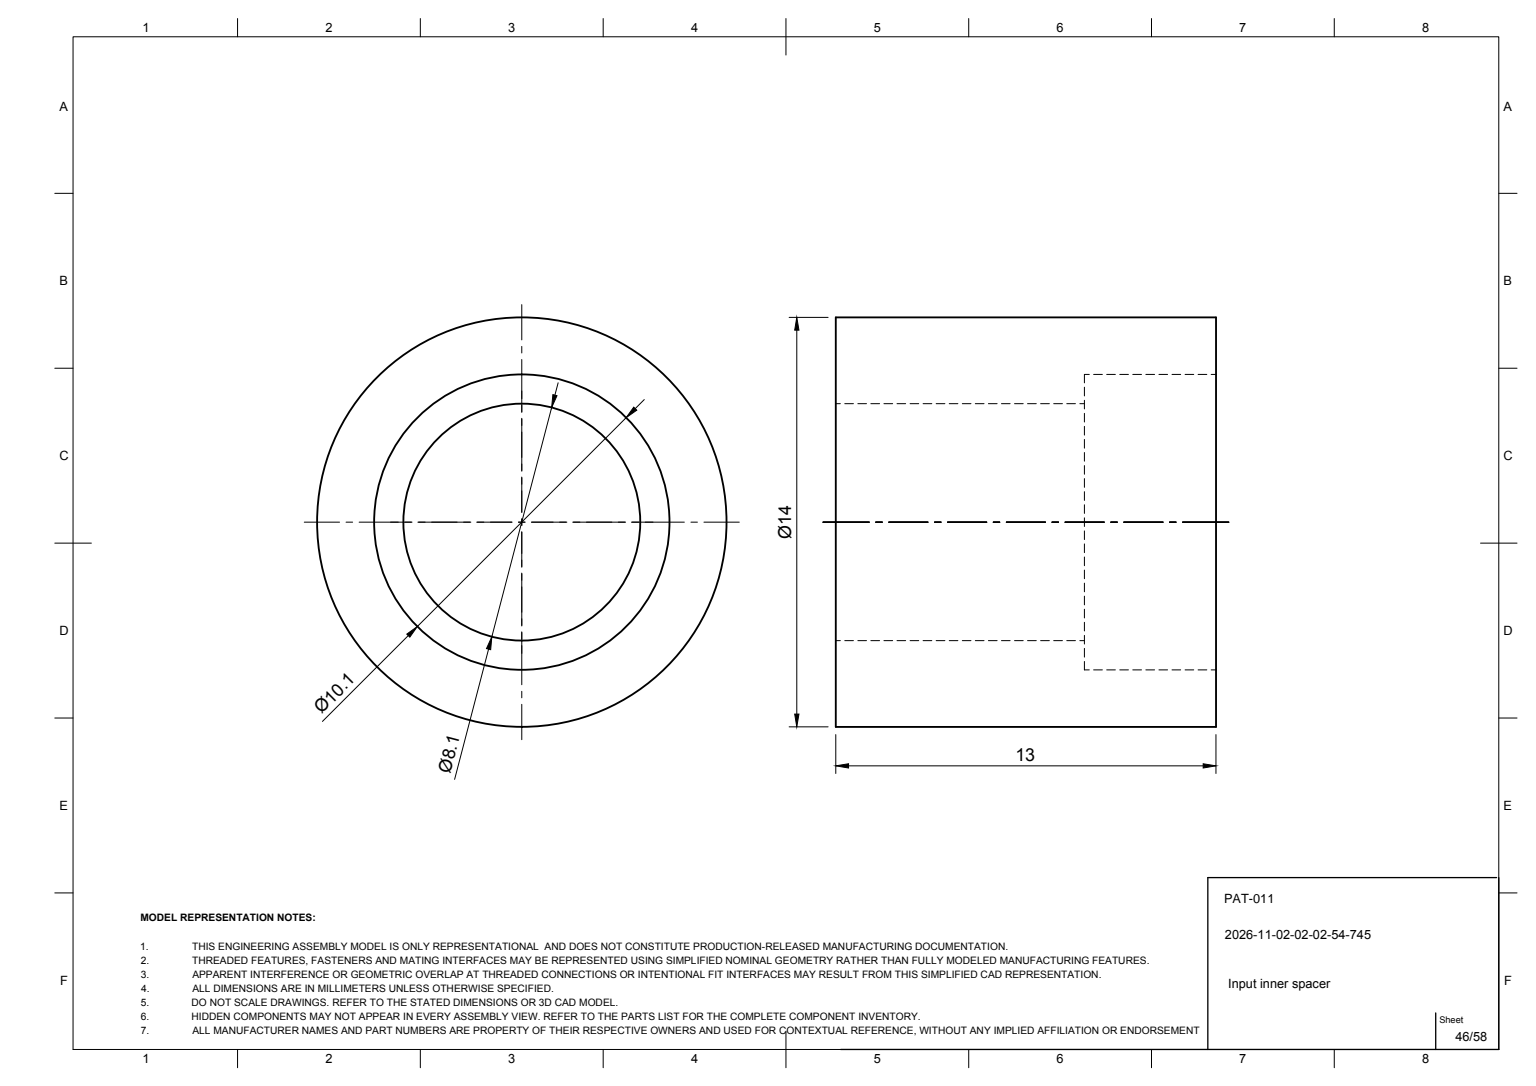
ISO-10303-21;
HEADER;
/* Generated by software containing ST-Developer
 * from STEP Tools, Inc. (www.steptools.com) 
 */

FILE_DESCRIPTION(
/* description */ ('Belt tension measurement rig'),
/* implementation_level */ '2;1');

FILE_NAME(
/* name */ 'Input inner spacer.step',
/* time_stamp */ '2026-10-28T03:24:44-07:00',
/* author */ (''),
/* organization */ (''),
/* preprocessor_version */ 'ST-DEVELOPER v20.2',
/* originating_system */ 'Autodesk Translation Framework v15.17.0.0',
/* authorisation */ '');

FILE_SCHEMA (('AUTOMOTIVE_DESIGN { 1 0 10303 214 3 1 1 }'));
ENDSEC;

DATA;
#10=MECHANICAL_DESIGN_GEOMETRIC_PRESENTATION_REPRESENTATION('',(#745),#23587);
#620=SHAPE_REPRESENTATION_RELATIONSHIP('SRR','None',#23870,#675);
#675=ADVANCED_BREP_SHAPE_REPRESENTATION('',(#813),#23568);
#745=STYLED_ITEM('',(#24225),#813);
#813=MANIFOLD_SOLID_BREP('Body1',#12252);
#988=FACE_BOUND('',#2675,.T.);
#989=FACE_BOUND('',#2679,.T.);
#990=FACE_BOUND('',#2681,.T.);
#1283=PLANE('',#13832);
#1284=PLANE('',#13839);
#1285=PLANE('',#13840);
#1810=FACE_OUTER_BOUND('',#2673,.T.);
#1811=FACE_OUTER_BOUND('',#2674,.T.);
#1812=FACE_OUTER_BOUND('',#2676,.T.);
#1813=FACE_OUTER_BOUND('',#2677,.T.);
#1814=FACE_OUTER_BOUND('',#2678,.T.);
#1815=FACE_OUTER_BOUND('',#2680,.T.);
#2673=EDGE_LOOP('',(#9950,#9951,#9952,#9953));
#2674=EDGE_LOOP('',(#9954));
#2675=EDGE_LOOP('',(#9955));
#2676=EDGE_LOOP('',(#9956,#9957,#9958,#9959));
#2677=EDGE_LOOP('',(#9960,#9961,#9962,#9963));
#2678=EDGE_LOOP('',(#9964));
#2679=EDGE_LOOP('',(#9965));
#2680=EDGE_LOOP('',(#9966));
#2681=EDGE_LOOP('',(#9967));
#3498=LINE('',#21484,#4249);
#3499=LINE('',#21491,#4250);
#3500=LINE('',#21497,#4251);
#4249=VECTOR('',#16957,0.505);
#4250=VECTOR('',#16966,0.405);
#4251=VECTOR('',#16973,0.7);
#4906=CIRCLE('',#13830,0.505);
#4907=CIRCLE('',#13831,0.505);
#4908=CIRCLE('',#13833,0.405);
#4909=CIRCLE('',#13835,0.405);
#4910=CIRCLE('',#13837,0.7);
#4911=CIRCLE('',#13838,0.7);
#5921=VERTEX_POINT('',#21481);
#5922=VERTEX_POINT('',#21483);
#5923=VERTEX_POINT('',#21487);
#5924=VERTEX_POINT('',#21490);
#5925=VERTEX_POINT('',#21494);
#5926=VERTEX_POINT('',#21496);
#7334=EDGE_CURVE('',#5921,#5921,#4906,.T.);
#7335=EDGE_CURVE('',#5921,#5922,#3498,.T.);
#7336=EDGE_CURVE('',#5922,#5922,#4907,.T.);
#7337=EDGE_CURVE('',#5923,#5923,#4908,.T.);
#7338=EDGE_CURVE('',#5923,#5924,#3499,.T.);
#7339=EDGE_CURVE('',#5924,#5924,#4909,.T.);
#7340=EDGE_CURVE('',#5925,#5925,#4910,.T.);
#7341=EDGE_CURVE('',#5925,#5926,#3500,.T.);
#7342=EDGE_CURVE('',#5926,#5926,#4911,.T.);
#9950=ORIENTED_EDGE('',*,*,#7334,.F.);
#9951=ORIENTED_EDGE('',*,*,#7335,.T.);
#9952=ORIENTED_EDGE('',*,*,#7336,.F.);
#9953=ORIENTED_EDGE('',*,*,#7335,.F.);
#9954=ORIENTED_EDGE('',*,*,#7334,.T.);
#9955=ORIENTED_EDGE('',*,*,#7337,.F.);
#9956=ORIENTED_EDGE('',*,*,#7337,.T.);
#9957=ORIENTED_EDGE('',*,*,#7338,.T.);
#9958=ORIENTED_EDGE('',*,*,#7339,.T.);
#9959=ORIENTED_EDGE('',*,*,#7338,.F.);
#9960=ORIENTED_EDGE('',*,*,#7340,.F.);
#9961=ORIENTED_EDGE('',*,*,#7341,.T.);
#9962=ORIENTED_EDGE('',*,*,#7342,.T.);
#9963=ORIENTED_EDGE('',*,*,#7341,.F.);
#9964=ORIENTED_EDGE('',*,*,#7340,.T.);
#9965=ORIENTED_EDGE('',*,*,#7336,.T.);
#9966=ORIENTED_EDGE('',*,*,#7342,.F.);
#9967=ORIENTED_EDGE('',*,*,#7339,.F.);
#11322=CYLINDRICAL_SURFACE('',#13829,0.505);
#11323=CYLINDRICAL_SURFACE('',#13834,0.405);
#11324=CYLINDRICAL_SURFACE('',#13836,0.7);
#11951=ADVANCED_FACE('',(#1810),#11322,.F.);
#11952=ADVANCED_FACE('',(#1811,#988),#1283,.T.);
#11953=ADVANCED_FACE('',(#1812),#11323,.F.);
#11954=ADVANCED_FACE('',(#1813),#11324,.T.);
#11955=ADVANCED_FACE('',(#1814,#989),#1284,.T.);
#11956=ADVANCED_FACE('',(#1815,#990),#1285,.F.);
#12252=CLOSED_SHELL('',(#11951,#11952,#11953,#11954,#11955,#11956));
#13828=AXIS2_PLACEMENT_3D('',#21479,#16951,#16952);
#13829=AXIS2_PLACEMENT_3D('',#21480,#16953,#16954);
#13830=AXIS2_PLACEMENT_3D('',#21482,#16955,#16956);
#13831=AXIS2_PLACEMENT_3D('',#21485,#16958,#16959);
#13832=AXIS2_PLACEMENT_3D('',#21486,#16960,#16961);
#13833=AXIS2_PLACEMENT_3D('',#21488,#16962,#16963);
#13834=AXIS2_PLACEMENT_3D('',#21489,#16964,#16965);
#13835=AXIS2_PLACEMENT_3D('',#21492,#16967,#16968);
#13836=AXIS2_PLACEMENT_3D('',#21493,#16969,#16970);
#13837=AXIS2_PLACEMENT_3D('',#21495,#16971,#16972);
#13838=AXIS2_PLACEMENT_3D('',#21498,#16974,#16975);
#13839=AXIS2_PLACEMENT_3D('',#21499,#16976,#16977);
#13840=AXIS2_PLACEMENT_3D('',#21500,#16978,#16979);
#16951=DIRECTION('axis',(0.,0.,1.));
#16952=DIRECTION('refdir',(1.,0.,0.));
#16953=DIRECTION('center_axis',(0.,1.,0.));
#16954=DIRECTION('ref_axis',(1.,0.,0.));
#16955=DIRECTION('center_axis',(0.,1.,0.));
#16956=DIRECTION('ref_axis',(1.,0.,0.));
#16957=DIRECTION('',(0.,1.,0.));
#16958=DIRECTION('center_axis',(0.,-1.,0.));
#16959=DIRECTION('ref_axis',(1.,0.,0.));
#16960=DIRECTION('center_axis',(0.,1.,0.));
#16961=DIRECTION('ref_axis',(1.,0.,0.));
#16962=DIRECTION('center_axis',(0.,1.,0.));
#16963=DIRECTION('ref_axis',(1.,0.,0.));
#16964=DIRECTION('center_axis',(0.,1.,0.));
#16965=DIRECTION('ref_axis',(1.,0.,0.));
#16966=DIRECTION('',(0.,-1.,0.));
#16967=DIRECTION('center_axis',(0.,-1.,0.));
#16968=DIRECTION('ref_axis',(1.,0.,0.));
#16969=DIRECTION('center_axis',(0.,1.,0.));
#16970=DIRECTION('ref_axis',(1.,0.,0.));
#16971=DIRECTION('center_axis',(0.,1.,0.));
#16972=DIRECTION('ref_axis',(1.,0.,0.));
#16973=DIRECTION('',(0.,-1.,0.));
#16974=DIRECTION('center_axis',(0.,1.,0.));
#16975=DIRECTION('ref_axis',(1.,0.,0.));
#16976=DIRECTION('center_axis',(0.,1.,0.));
#16977=DIRECTION('ref_axis',(1.,0.,0.));
#16978=DIRECTION('center_axis',(0.,1.,0.));
#16979=DIRECTION('ref_axis',(1.,0.,0.));
#21479=CARTESIAN_POINT('',(0.,0.,0.));
#21480=CARTESIAN_POINT('Origin',(0.,-1.8,7.));
#21481=CARTESIAN_POINT('',(-0.505,-1.8,7.));
#21482=CARTESIAN_POINT('Origin',(0.,-1.8,7.));
#21483=CARTESIAN_POINT('',(-0.505,-1.35,7.));
#21484=CARTESIAN_POINT('',(-0.505,-1.8,7.));
#21485=CARTESIAN_POINT('Origin',(0.,-1.35,7.));
#21486=CARTESIAN_POINT('Origin',(0.,-1.8,7.));
#21487=CARTESIAN_POINT('',(-0.405,-1.8,7.));
#21488=CARTESIAN_POINT('Origin',(0.,-1.8,7.));
#21489=CARTESIAN_POINT('Origin',(0.,-2.65,7.));
#21490=CARTESIAN_POINT('',(-0.405,-2.65,7.));
#21491=CARTESIAN_POINT('',(-0.405,-2.65,7.));
#21492=CARTESIAN_POINT('Origin',(0.,-2.65,7.));
#21493=CARTESIAN_POINT('Origin',(0.,-2.65,7.));
#21494=CARTESIAN_POINT('',(-0.7,-1.35,7.));
#21495=CARTESIAN_POINT('Origin',(0.,-1.35,7.));
#21496=CARTESIAN_POINT('',(-0.7,-2.65,7.));
#21497=CARTESIAN_POINT('',(-0.7,-2.65,7.));
#21498=CARTESIAN_POINT('Origin',(0.,-2.65,7.));
#21499=CARTESIAN_POINT('Origin',(0.,-1.35,7.));
#21500=CARTESIAN_POINT('Origin',(0.,-2.65,7.));
#23503=UNCERTAINTY_MEASURE_WITH_UNIT(LENGTH_MEASURE(0.001),#23588,
'DISTANCE_ACCURACY_VALUE',
'Maximum model space distance between geometric entities at asserted c
onnectivities');
#23522=UNCERTAINTY_MEASURE_WITH_UNIT(LENGTH_MEASURE(0.001),#23588,
'DISTANCE_ACCURACY_VALUE',
'Maximum model space distance between geometric entities at asserted c
onnectivities');
#23568=(
GEOMETRIC_REPRESENTATION_CONTEXT(3)
GLOBAL_UNCERTAINTY_ASSIGNED_CONTEXT((#23503))
GLOBAL_UNIT_ASSIGNED_CONTEXT((#23588,#23590,#23591))
REPRESENTATION_CONTEXT('','3D')
);
#23587=(
GEOMETRIC_REPRESENTATION_CONTEXT(3)
GLOBAL_UNCERTAINTY_ASSIGNED_CONTEXT((#23522))
GLOBAL_UNIT_ASSIGNED_CONTEXT((#23588,#23590,#23591))
REPRESENTATION_CONTEXT('','3D')
);
#23588=(
LENGTH_UNIT()
NAMED_UNIT(*)
SI_UNIT(.CENTI.,.METRE.)
);
#23590=(
NAMED_UNIT(*)
PLANE_ANGLE_UNIT()
SI_UNIT($,.RADIAN.)
);
#23591=(
NAMED_UNIT(*)
SI_UNIT($,.STERADIAN.)
SOLID_ANGLE_UNIT()
);
#23637=SHAPE_DEFINITION_REPRESENTATION(#23714,#23870);
#23714=PRODUCT_DEFINITION_SHAPE('',$,#23935);
#23870=SHAPE_REPRESENTATION('',(#13828),#23568);
#23889=PRODUCT_DEFINITION_CONTEXT('part definition',#24083,'design');
#23935=PRODUCT_DEFINITION('Input inner spacer','Input inner spacer',#23999,
#23889);
#23999=PRODUCT_DEFINITION_FORMATION('',$,#24130);
#24083=APPLICATION_CONTEXT(
'Core Data for Automotive Mechanical Design Process');
#24084=PRODUCT_CONTEXT('part definition',#24083,'mechanical');
#24130=PRODUCT('Input inner spacer','Input inner spacer',
'Input inner spacer',(#24084));
#24219=COLOUR_RGB('Off White',0.89,0.88,0.83);
#24220=FILL_AREA_STYLE_COLOUR('',#24219);
#24221=FILL_AREA_STYLE('',(#24220));
#24222=SURFACE_STYLE_FILL_AREA(#24221);
#24223=SURFACE_SIDE_STYLE('',(#24222));
#24224=SURFACE_STYLE_USAGE(.BOTH.,#24223);
#24225=PRESENTATION_STYLE_ASSIGNMENT((#24224));
ENDSEC;
END-ISO-10303-21;
